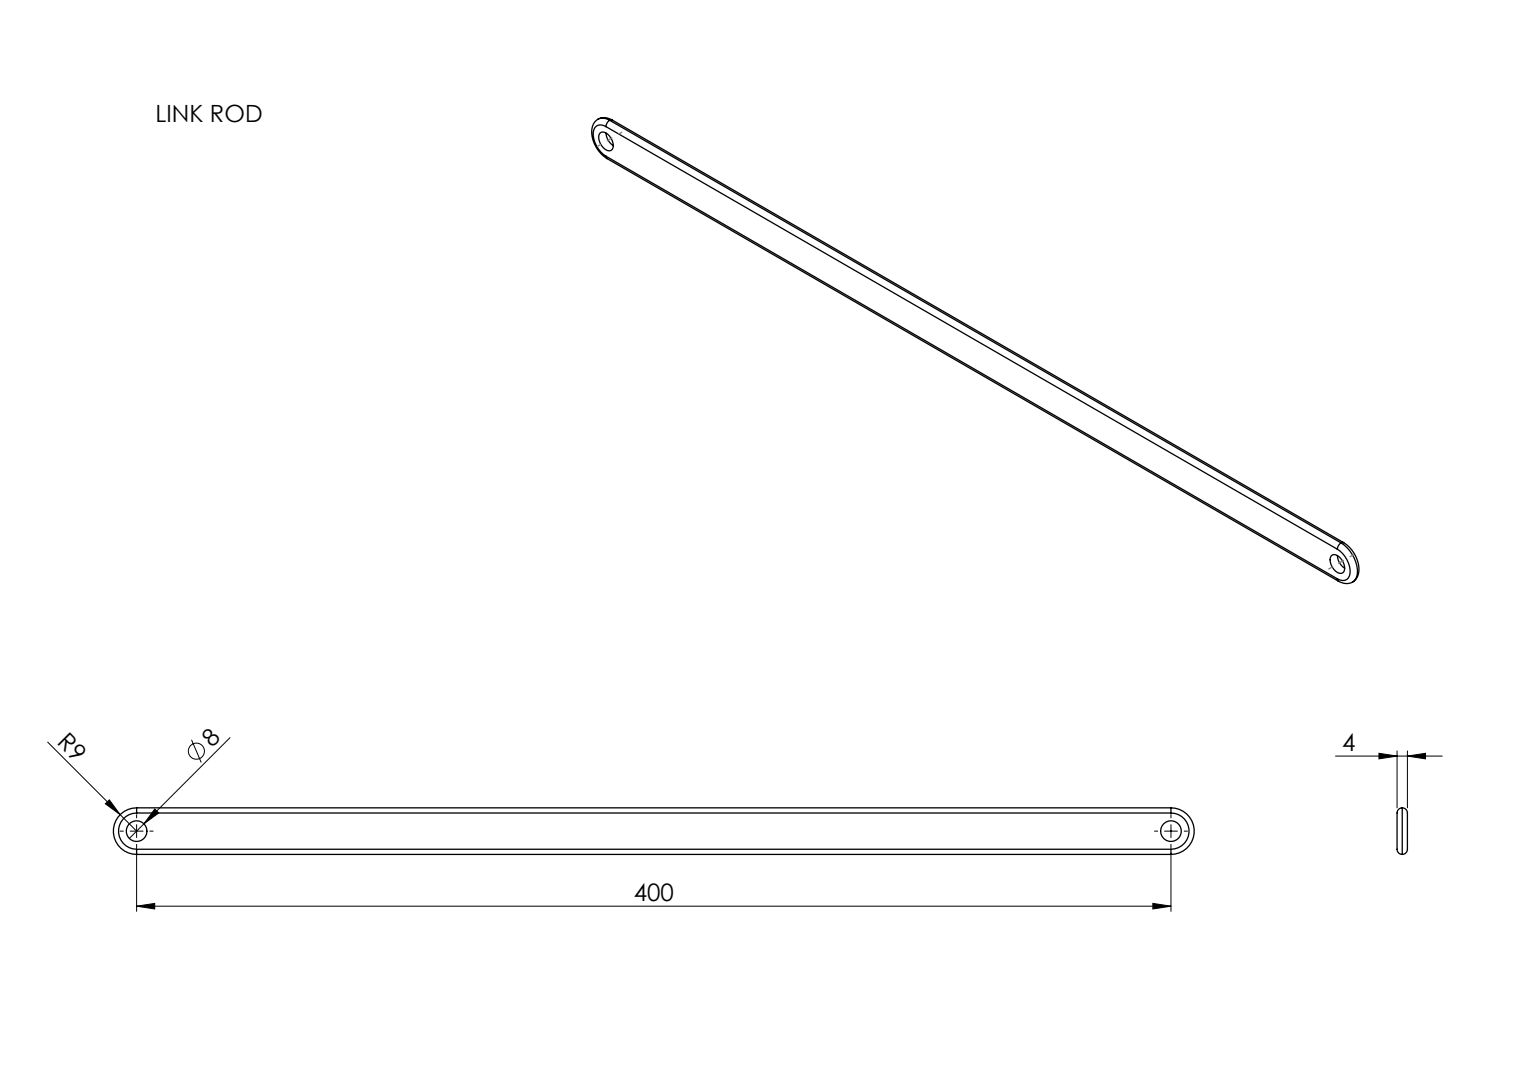
ISO-10303-21;
HEADER;
FILE_DESCRIPTION (('STEP AP214'),
    '1' );
FILE_NAME ('link rod.step',
    '2026-09-30T16:28:02',
    ( '' ),
    ( '' ),
    'SwSTEP 2.0',
    'SolidWorks 2026',
    '' );
FILE_SCHEMA (( 'AUTOMOTIVE_DESIGN' ));
ENDSEC;

DATA;
#66=CARTESIAN_POINT ( 'NONE',  ( 16.00000000000017053, 34.64101615137744972, 14.00000000000000178 ) ) ;
#129=ORIENTED_EDGE ( 'NONE', *, *, #17959, .T. ) ;
#135=ADVANCED_FACE ( 'NONE', ( #10257 ), #20396, .T. ) ;
#175=EDGE_CURVE ( 'NONE', #8969, #15955, #19420, .T. ) ;
#310=CARTESIAN_POINT ( 'NONE',  ( 20.00000000000017053, 34.64101615137744972, 14.00000000000000178 ) ) ;
#392=AXIS2_PLACEMENT_3D ( 'NONE', #4305, #4004, #27842 ) ;
#428=DIRECTION ( 'NONE',  ( -0.000000000000000000, -0.000000000000000000, -1.000000000000000000 ) ) ;
#440=AXIS2_PLACEMENT_3D ( 'NONE', #10772, #20082, #29458 ) ;
#528=( NAMED_UNIT ( * ) SI_UNIT ( $, .STERADIAN. ) SOLID_ANGLE_UNIT ( ) );
#621=CARTESIAN_POINT ( 'NONE',  ( 416.0000000000002274, 34.64101615137744972, 14.00000000000000178 ) ) ;
#662=EDGE_LOOP ( 'NONE', ( #30038, #11644, #23930, #20941 ) ) ;
#674=EDGE_LOOP ( 'NONE', ( #23723, #129, #3090, #8885 ) ) ;
#713=EDGE_CURVE ( 'NONE', #23249, #7514, #4350, .T. ) ;
#774=PRODUCT_CONTEXT ( 'NONE', #9279, 'mechanical' ) ;
#794=ORIENTED_EDGE ( 'NONE', *, *, #25575, .T. ) ;
#849=AXIS2_PLACEMENT_3D ( 'NONE', #1764, #20801, #6484 ) ;
#864=ADVANCED_FACE ( 'NONE', ( #26946 ), #28757, .T. ) ;
#870=VECTOR ( 'NONE', #18675, 1000.000000000000000 ) ;
#1083=DIRECTION ( 'NONE',  ( -0.000000000000000000, -0.000000000000000000, -1.000000000000000000 ) ) ;
#1179=DIRECTION ( 'NONE',  ( 1.000000000000000000, 0.000000000000000000, 0.000000000000000000 ) ) ;
#1186=CARTESIAN_POINT ( 'NONE',  ( 20.00000000000017053, 34.64101615137744972, 10.00000000000000178 ) ) ;
#1233=FACE_OUTER_BOUND ( 'NONE', #4292, .T. ) ;
#1344=DIRECTION ( 'NONE',  ( 1.000000000000000000, -0.000000000000000000, -0.000000000000000000 ) ) ;
#1401=DIRECTION ( 'NONE',  ( 0.000000000000000000, 0.000000000000000000, 1.000000000000000000 ) ) ;
#1402=ORIENTED_EDGE ( 'NONE', *, *, #6678, .T. ) ;
#1466=CYLINDRICAL_SURFACE ( 'NONE', #4682, 2.000000000000000000 ) ;
#1628=ADVANCED_FACE ( 'NONE', ( #7128 ), #19463, .T. ) ;
#1649=CARTESIAN_POINT ( 'NONE',  ( 20.00000000000017053, 27.64101615137744972, 12.00000000000000178 ) ) ;
#1664=ORIENTED_EDGE ( 'NONE', *, *, #12629, .T. ) ;
#1764=CARTESIAN_POINT ( 'NONE',  ( 420.0000000000002274, 34.64101615137744972, 10.00000000000000178 ) ) ;
#1776=VECTOR ( 'NONE', #11033, 1000.000000000000000 ) ;
#1792=ORIENTED_EDGE ( 'NONE', *, *, #30164, .T. ) ;
#1813=CARTESIAN_POINT ( 'NONE',  ( 416.0000000000002274, 34.64101615137744972, 10.00000000000000178 ) ) ;
#1819=ORIENTED_EDGE ( 'NONE', *, *, #20781, .T. ) ;
#1876=SURFACE_SIDE_STYLE ('',( #27386 ) ) ;
#2221=FILL_AREA_STYLE ('',( #18679 ) ) ;
#2391=AXIS2_PLACEMENT_3D ( 'NONE', #310, #18914, #21646 ) ;
#2396=ORIENTED_EDGE ( 'NONE', *, *, #11470, .T. ) ;
#2428=CARTESIAN_POINT ( 'NONE',  ( 20.00000000000017053, 34.64101615137744972, 14.00000000000000178 ) ) ;
#2445=STYLED_ITEM ( 'NONE', ( #18984 ), #16384 ) ;
#2468=PRODUCT_DEFINITION_FORMATION_WITH_SPECIFIED_SOURCE ( 'ANY', '', #20070, .NOT_KNOWN. ) ;
#2584=DIRECTION ( 'NONE',  ( 0.000000000000000000, 0.000000000000000000, 1.000000000000000000 ) ) ;
#2603=AXIS2_PLACEMENT_3D ( 'NONE', #20401, #18720, #4388 ) ;
#2609=ORIENTED_EDGE ( 'NONE', *, *, #26221, .F. ) ;
#2624=VERTEX_POINT ( 'NONE', #7362 ) ;
#2662=EDGE_LOOP ( 'NONE', ( #12047, #2609 ) ) ;
#2912=DIRECTION ( 'NONE',  ( -1.000000000000000000, 0.000000000000000000, 0.000000000000000000 ) ) ;
#3024=CARTESIAN_POINT ( 'NONE',  ( 427.0000000000002274, 34.64101615137744972, 14.00000000000000178 ) ) ;
#3081=ORIENTED_EDGE ( 'NONE', *, *, #17585, .T. ) ;
#3090=ORIENTED_EDGE ( 'NONE', *, *, #25828, .T. ) ;
#3122=CARTESIAN_POINT ( 'NONE',  ( 416.0000000000002274, 34.64101615137744972, 14.00000000000000178 ) ) ;
#3146=CARTESIAN_POINT ( 'NONE',  ( 420.0000000000002274, 34.64101615137744972, 12.00000000000000178 ) ) ;
#3242=ADVANCED_FACE ( 'NONE', ( #21504, #17633, #24672 ), #26248, .T. ) ;
#3383=DIRECTION ( 'NONE',  ( 1.000000000000000000, -0.000000000000000000, 0.000000000000000000 ) ) ;
#3440=EDGE_CURVE ( 'NONE', #8350, #23249, #13584, .T. ) ;
#3539=LINE ( 'NONE', #22146, #28159 ) ;
#3588=CARTESIAN_POINT ( 'NONE',  ( 420.0000000000002274, 34.64101615137744972, 12.00000000000000178 ) ) ;
#3601=CARTESIAN_POINT ( 'NONE',  ( 429.0000000000002274, 34.64101615137744972, 12.00000000000000178 ) ) ;
#3646=EDGE_CURVE ( 'NONE', #28740, #7514, #22998, .T. ) ;
#3694=ORIENTED_EDGE ( 'NONE', *, *, #15888, .T. ) ;
#3736=ORIENTED_EDGE ( 'NONE', *, *, #11470, .F. ) ;
#3777=DIRECTION ( 'NONE',  ( 1.000000000000000000, 0.000000000000000000, 0.000000000000000000 ) ) ;
#3861=AXIS2_PLACEMENT_3D ( 'NONE', #3146, #5571, #17603 ) ;
#4004=DIRECTION ( 'NONE',  ( 0.000000000000000000, 0.000000000000000000, 1.000000000000000000 ) ) ;
#4060=DIRECTION ( 'NONE',  ( 0.000000000000000000, 0.000000000000000000, -1.000000000000000000 ) ) ;
#4128=LINE ( 'NONE', #17840, #13960 ) ;
#4196=TOROIDAL_SURFACE ( 'NONE', #5144, 7.000000000000000888, 2.000000000000000000 ) ;
#4259=COLOUR_RGB ( '', 0.08235294, 0.09019608, 0.10196078) ;
#4292=EDGE_LOOP ( 'NONE', ( #1664, #4911, #6108, #16603 ) ) ;
#4305=CARTESIAN_POINT ( 'NONE',  ( 420.0000000000002274, 34.64101615137744972, 14.00000000000000178 ) ) ;
#4306=DIRECTION ( 'NONE',  ( 1.000000000000000000, 0.000000000000000000, 0.000000000000000000 ) ) ;
#4350=CIRCLE ( 'NONE', #3861, 9.000000000000007105 ) ;
#4388=DIRECTION ( 'NONE',  ( 0.000000000000000000, 0.000000000000000000, 1.000000000000000000 ) ) ;
#4539=DIRECTION ( 'NONE',  ( 0.000000000000000000, 0.000000000000000000, 1.000000000000000000 ) ) ;
#4541=CIRCLE ( 'NONE', #9384, 2.000000000000000000 ) ;
#4640=SHAPE_REPRESENTATION_RELATIONSHIP ( 'NONE' , 'NONE' ,  #19847, #16384 ) ;
#4682=AXIS2_PLACEMENT_3D ( 'NONE', #22519, #24507, #24965 ) ;
#4821=ORIENTED_EDGE ( 'NONE', *, *, #25575, .F. ) ;
#4904=CIRCLE ( 'NONE', #20492, 2.000000000000000000 ) ;
#4911=ORIENTED_EDGE ( 'NONE', *, *, #9408, .F. ) ;
#4940=( LENGTH_UNIT ( ) NAMED_UNIT ( * ) SI_UNIT ( .MILLI., .METRE. ) );
#4992=EDGE_LOOP ( 'NONE', ( #20045, #15327, #18477, #14680 ) ) ;
#5028=CARTESIAN_POINT ( 'NONE',  ( 20.00000000000017053, 34.64101615137744972, 14.00000000000000178 ) ) ;
#5144=AXIS2_PLACEMENT_3D ( 'NONE', #16753, #26076, #26228 ) ;
#5185=ORIENTED_EDGE ( 'NONE', *, *, #3646, .T. ) ;
#5247=VERTEX_POINT ( 'NONE', #18395 ) ;
#5272=ORIENTED_EDGE ( 'NONE', *, *, #9408, .T. ) ;
#5360=VECTOR ( 'NONE', #25155, 1000.000000000000000 ) ;
#5435=CARTESIAN_POINT ( 'NONE',  ( 0.000000000000000000, 0.000000000000000000, 0.000000000000000000 ) ) ;
#5447=DIRECTION ( 'NONE',  ( 0.000000000000000000, 0.000000000000000000, -1.000000000000000000 ) ) ;
#5537=DIRECTION ( 'NONE',  ( 1.000000000000000000, 0.000000000000000000, 0.000000000000000000 ) ) ;
#5571=DIRECTION ( 'NONE',  ( -0.000000000000000000, -0.000000000000000000, -1.000000000000000000 ) ) ;
#5577=CARTESIAN_POINT ( 'NONE',  ( 420.0000000000002274, 34.64101615137744972, 14.00000000000000178 ) ) ;
#5614=ORIENTED_EDGE ( 'NONE', *, *, #6819, .F. ) ;
#5618=VERTEX_POINT ( 'NONE', #22506 ) ;
#5628=CARTESIAN_POINT ( 'NONE',  ( 20.00000000000017053, 25.64101615137744616, 12.00000000000000178 ) ) ;
#5735=CARTESIAN_POINT ( 'NONE',  ( 20.00000000000017053, 34.64101615137744972, 10.00000000000000178 ) ) ;
#5886=EDGE_LOOP ( 'NONE', ( #16599, #6085, #10247, #2396 ) ) ;
#5903=DIRECTION ( 'NONE',  ( 1.000000000000000000, 0.000000000000000000, 0.000000000000000000 ) ) ;
#5922=ORIENTED_EDGE ( 'NONE', *, *, #25828, .F. ) ;
#6003=DIRECTION ( 'NONE',  ( 1.000000000000000000, 0.000000000000000000, 0.000000000000000000 ) ) ;
#6085=ORIENTED_EDGE ( 'NONE', *, *, #17585, .F. ) ;
#6102=ORIENTED_EDGE ( 'NONE', *, *, #9626, .T. ) ;
#6108=ORIENTED_EDGE ( 'NONE', *, *, #24279, .F. ) ;
#6142=AXIS2_PLACEMENT_3D ( 'NONE', #5028, #12042, #2912 ) ;
#6191=ADVANCED_FACE ( 'NONE', ( #10705, #13294, #15729 ), #10546, .F. ) ;
#6223=AXIS2_PLACEMENT_3D ( 'NONE', #12751, #17037, #5447 ) ;
#6248=TOROIDAL_SURFACE ( 'NONE', #13052, 7.000000000000000888, 2.000000000000000000 ) ;
#6258=VERTEX_POINT ( 'NONE', #15118 ) ;
#6275=ORIENTED_EDGE ( 'NONE', *, *, #21485, .T. ) ;
#6292=CARTESIAN_POINT ( 'NONE',  ( 20.00000000000017053, 34.64101615137744972, 12.00000000000000178 ) ) ;
#6393=DIRECTION ( 'NONE',  ( -1.000000000000000000, 0.000000000000000000, 0.000000000000000000 ) ) ;
#6484=DIRECTION ( 'NONE',  ( 1.000000000000000000, 0.000000000000000000, 0.000000000000000000 ) ) ;
#6566=DIRECTION ( 'NONE',  ( -0.000000000000000000, -0.000000000000000000, -1.000000000000000000 ) ) ;
#6678=EDGE_CURVE ( 'NONE', #7514, #9503, #6876, .T. ) ;
#6728=DIRECTION ( 'NONE',  ( -0.000000000000000000, -0.000000000000000000, -1.000000000000000000 ) ) ;
#6737=( NAMED_UNIT ( * ) SI_UNIT ( $, .STERADIAN. ) SOLID_ANGLE_UNIT ( ) );
#6770=DIRECTION ( 'NONE',  ( -1.000000000000000000, 0.000000000000000000, -0.000000000000000000 ) ) ;
#6819=EDGE_CURVE ( 'NONE', #8969, #24258, #4904, .T. ) ;
#6850=CARTESIAN_POINT ( 'NONE',  ( 24.00000000000017053, 34.64101615137744972, 10.00000000000000178 ) ) ;
#6874=DIRECTION ( 'NONE',  ( -1.000000000000000000, 0.000000000000000000, 0.000000000000000000 ) ) ;
#6876=CIRCLE ( 'NONE', #23944, 2.000000000000000000 ) ;
#6905=DIRECTION ( 'NONE',  ( 0.000000000000000000, 0.000000000000000000, 1.000000000000000000 ) ) ;
#6940=( NAMED_UNIT ( * ) PLANE_ANGLE_UNIT ( ) SI_UNIT ( $, .RADIAN. ) );
#6982=ORIENTED_EDGE ( 'NONE', *, *, #3646, .F. ) ;
#7034=EDGE_LOOP ( 'NONE', ( #15544, #8379, #5614, #28228 ) ) ;
#7111=AXIS2_PLACEMENT_3D ( 'NONE', #9110, #2584, #18740 ) ;
#7128=FACE_OUTER_BOUND ( 'NONE', #7034, .T. ) ;
#7210=CIRCLE ( 'NONE', #10130, 7.000000000000006217 ) ;
#7298=FACE_OUTER_BOUND ( 'NONE', #19832, .T. ) ;
#7334=VERTEX_POINT ( 'NONE', #13192 ) ;
#7357=ORIENTED_EDGE ( 'NONE', *, *, #25373, .T. ) ;
#7362=CARTESIAN_POINT ( 'NONE',  ( 420.0000000000002274, 27.64101615137744972, 14.00000000000000178 ) ) ;
#7514=VERTEX_POINT ( 'NONE', #3601 ) ;
#7683=AXIS2_PLACEMENT_3D ( 'NONE', #10441, #17464, #10754 ) ;
#7769=DIRECTION ( 'NONE',  ( 0.000000000000000000, 0.000000000000000000, -1.000000000000000000 ) ) ;
#7795=DIRECTION ( 'NONE',  ( -1.000000000000000000, 0.000000000000000000, 0.000000000000000000 ) ) ;
#7964=CARTESIAN_POINT ( 'NONE',  ( 20.00000000000017053, 27.64101615137744972, 10.00000000000000178 ) ) ;
#7972=DIRECTION ( 'NONE',  ( 0.000000000000000000, 0.000000000000000000, 1.000000000000000000 ) ) ;
#8107=DIRECTION ( 'NONE',  ( 1.000000000000000000, 0.000000000000000000, -0.000000000000000000 ) ) ;
#8142=CYLINDRICAL_SURFACE ( 'NONE', #21760, 2.000000000000000000 ) ;
#8147=MECHANICAL_DESIGN_GEOMETRIC_PRESENTATION_REPRESENTATION('',(#28653),#25224);
#8230=DIRECTION ( 'NONE',  ( 0.000000000000000000, 0.000000000000000000, -1.000000000000000000 ) ) ;
#8350=VERTEX_POINT ( 'NONE', #18795 ) ;
#8379=ORIENTED_EDGE ( 'NONE', *, *, #29365, .F. ) ;
#8542=EDGE_CURVE ( 'NONE', #16524, #12515, #20589, .T. ) ;
#8639=DIRECTION ( 'NONE',  ( 0.000000000000000000, 0.000000000000000000, -1.000000000000000000 ) ) ;
#8841=CARTESIAN_POINT ( 'NONE',  ( 420.0000000000002274, 34.64101615137744972, 10.00000000000000178 ) ) ;
#8874=AXIS2_PLACEMENT_3D ( 'NONE', #15740, #9009, #4306 ) ;
#8885=ORIENTED_EDGE ( 'NONE', *, *, #25484, .F. ) ;
#8909=ORIENTED_EDGE ( 'NONE', *, *, #3440, .F. ) ;
#8915=DIRECTION ( 'NONE',  ( 1.000000000000000000, 0.000000000000000000, -0.000000000000000000 ) ) ;
#8969=VERTEX_POINT ( 'NONE', #5628 ) ;
#9009=DIRECTION ( 'NONE',  ( 0.000000000000000000, 0.000000000000000000, 1.000000000000000000 ) ) ;
#9027=ORIENTED_EDGE ( 'NONE', *, *, #19612, .F. ) ;
#9058=EDGE_CURVE ( 'NONE', #13389, #15955, #4541, .T. ) ;
#9059=CARTESIAN_POINT ( 'NONE',  ( 20.00000000000017053, 27.64101615137744972, 12.00000000000000178 ) ) ;
#9110=CARTESIAN_POINT ( 'NONE',  ( 420.0000000000002274, 34.64101615137744972, 14.00000000000000178 ) ) ;
#9122=CARTESIAN_POINT ( 'NONE',  ( 420.0000000000002274, 34.64101615137744972, 12.00000000000000178 ) ) ;
#9185=LINE ( 'NONE', #13182, #22046 ) ;
#9279=APPLICATION_CONTEXT ( 'automotive_design' ) ;
#9292=ORIENTED_EDGE ( 'NONE', *, *, #26050, .T. ) ;
#9331=ADVANCED_FACE ( 'NONE', ( #18269 ), #27778, .F. ) ;
#9384=AXIS2_PLACEMENT_3D ( 'NONE', #10531, #3383, #19839 ) ;
#9408=EDGE_CURVE ( 'NONE', #5618, #15809, #22720, .T. ) ;
#9503=VERTEX_POINT ( 'NONE', #3024 ) ;
#9564=ORIENTED_EDGE ( 'NONE', *, *, #12629, .F. ) ;
#9626=EDGE_CURVE ( 'NONE', #5247, #29002, #9734, .T. ) ;
#9729=CARTESIAN_POINT ( 'NONE',  ( 20.00000000000017053, 34.64101615137744972, 12.00000000000000178 ) ) ;
#9734=CIRCLE ( 'NONE', #22414, 4.000000000000000000 ) ;
#9757=CARTESIAN_POINT ( 'NONE',  ( 424.0000000000002274, 34.64101615137744972, 14.00000000000000178 ) ) ;
#9814=SURFACE_STYLE_USAGE ( .BOTH. , #23410 ) ;
#9997=CIRCLE ( 'NONE', #11456, 2.000000000000000000 ) ;
#10130=AXIS2_PLACEMENT_3D ( 'NONE', #26774, #7972, #15131 ) ;
#10216=AXIS2_PLACEMENT_3D ( 'NONE', #2428, #428, #23315 ) ;
#10247=ORIENTED_EDGE ( 'NONE', *, *, #19312, .F. ) ;
#10257=FACE_OUTER_BOUND ( 'NONE', #13592, .T. ) ;
#10279=( GEOMETRIC_REPRESENTATION_CONTEXT ( 3 ) GLOBAL_UNCERTAINTY_ASSIGNED_CONTEXT ( ( #17738 ) ) GLOBAL_UNIT_ASSIGNED_CONTEXT ( ( #18528, #6940, #26014 ) ) REPRESENTATION_CONTEXT ( 'NONE', 'WORKASPACE' ) );
#10441=CARTESIAN_POINT ( 'NONE',  ( 420.0000000000002274, 34.64101615137744972, 14.00000000000000178 ) ) ;
#10446=DIRECTION ( 'NONE',  ( 1.000000000000000000, 0.000000000000000000, 0.000000000000000000 ) ) ;
#10460=CARTESIAN_POINT ( 'NONE',  ( 20.00000000000017053, 34.64101615137744972, 10.00000000000000178 ) ) ;
#10531=CARTESIAN_POINT ( 'NONE',  ( 20.00000000000017053, 41.64101615137744972, 12.00000000000000178 ) ) ;
#10546=PLANE ( 'NONE',  #13206 ) ;
#10550=DIRECTION ( 'NONE',  ( 0.000000000000000000, 0.000000000000000000, -1.000000000000000000 ) ) ;
#10630=EDGE_LOOP ( 'NONE', ( #18972, #27063, #17217, #5922 ) ) ;
#10705=FACE_OUTER_BOUND ( 'NONE', #19796, .T. ) ;
#10750=CIRCLE ( 'NONE', #17557, 7.000000000000006217 ) ;
#10754=DIRECTION ( 'NONE',  ( -1.000000000000000000, 0.000000000000000000, 0.000000000000000000 ) ) ;
#10772=CARTESIAN_POINT ( 'NONE',  ( 420.0000000000002274, 41.64101615137744972, 12.00000000000000178 ) ) ;
#10830=AXIS2_PLACEMENT_3D ( 'NONE', #8841, #18001, #6874 ) ;
#11033=DIRECTION ( 'NONE',  ( 1.000000000000000000, -0.000000000000000000, -0.000000000000000000 ) ) ;
#11053=ORIENTED_EDGE ( 'NONE', *, *, #8542, .T. ) ;
#11158=ORIENTED_EDGE ( 'NONE', *, *, #8542, .F. ) ;
#11164=ORIENTED_EDGE ( 'NONE', *, *, #13444, .F. ) ;
#11165=DIRECTION ( 'NONE',  ( 1.000000000000000000, 0.000000000000000000, 0.000000000000000000 ) ) ;
#11179=AXIS2_PLACEMENT_3D ( 'NONE', #18871, #4539, #13829 ) ;
#11190=ORIENTED_EDGE ( 'NONE', *, *, #15589, .F. ) ;
#11325=UNCERTAINTY_MEASURE_WITH_UNIT (LENGTH_MEASURE( 1.000000000000000082E-05 ), #15429, 'distance_accuracy_value', 'NONE');
#11356=DIRECTION ( 'NONE',  ( 1.000000000000000000, 0.000000000000000000, 0.000000000000000000 ) ) ;
#11420=CIRCLE ( 'NONE', #24592, 2.000000000000000000 ) ;
#11456=AXIS2_PLACEMENT_3D ( 'NONE', #16778, #14319, #7769 ) ;
#11470=EDGE_CURVE ( 'NONE', #13296, #8969, #9185, .T. ) ;
#11498=CARTESIAN_POINT ( 'NONE',  ( 20.00000000000017053, 34.64101615137744972, 14.00000000000000178 ) ) ;
#11540=CARTESIAN_POINT ( 'NONE',  ( 420.0000000000002274, 34.64101615137744972, 14.00000000000000178 ) ) ;
#11644=ORIENTED_EDGE ( 'NONE', *, *, #713, .F. ) ;
#11840=MANIFOLD_SOLID_BREP ( 'Fillet1', #24820 ) ;
#12042=DIRECTION ( 'NONE',  ( -0.000000000000000000, -0.000000000000000000, -1.000000000000000000 ) ) ;
#12047=ORIENTED_EDGE ( 'NONE', *, *, #25373, .F. ) ;
#12149=DIRECTION ( 'NONE',  ( -1.000000000000000000, -0.000000000000000000, 0.000000000000000000 ) ) ;
#12225=( GEOMETRIC_REPRESENTATION_CONTEXT ( 3 ) GLOBAL_UNCERTAINTY_ASSIGNED_CONTEXT ( ( #15902 ) ) GLOBAL_UNIT_ASSIGNED_CONTEXT ( ( #4940, #20959, #528 ) ) REPRESENTATION_CONTEXT ( 'NONE', 'WORKASPACE' ) );
#12276=AXIS2_PLACEMENT_3D ( 'NONE', #21982, #14943, #7795 ) ;
#12479=CIRCLE ( 'NONE', #13937, 2.000000000000000000 ) ;
#12515=VERTEX_POINT ( 'NONE', #20424 ) ;
#12629=EDGE_CURVE ( 'NONE', #15955, #15809, #16953, .T. ) ;
#12678=FACE_OUTER_BOUND ( 'NONE', #20099, .T. ) ;
#12751=CARTESIAN_POINT ( 'NONE',  ( 20.00000000000017053, 41.64101615137744972, 12.00000000000000178 ) ) ;
#12803=EDGE_LOOP ( 'NONE', ( #7357, #1819, #11158, #11164 ) ) ;
#12826=CARTESIAN_POINT ( 'NONE',  ( 420.0000000000002274, 34.64101615137744972, 12.00000000000000178 ) ) ;
#13052=AXIS2_PLACEMENT_3D ( 'NONE', #6292, #6905, #11165 ) ;
#13129=ORIENTED_EDGE ( 'NONE', *, *, #23600, .T. ) ;
#13182=CARTESIAN_POINT ( 'NONE',  ( 20.00000000000017053, 25.64101615137744616, 12.00000000000000178 ) ) ;
#13190=AXIS2_PLACEMENT_3D ( 'NONE', #5435, #19606, #10446 ) ;
#13192=CARTESIAN_POINT ( 'NONE',  ( 20.00000000000017053, 27.64101615137744972, 14.00000000000000178 ) ) ;
#13206=AXIS2_PLACEMENT_3D ( 'NONE', #19704, #29068, #8107 ) ;
#13294=FACE_BOUND ( 'NONE', #28997, .T. ) ;
#13296=VERTEX_POINT ( 'NONE', #28429 ) ;
#13389=VERTEX_POINT ( 'NONE', #23821 ) ;
#13444=EDGE_CURVE ( 'NONE', #25744, #16524, #19663, .T. ) ;
#13500=VERTEX_POINT ( 'NONE', #9757 ) ;
#13584=CIRCLE ( 'NONE', #440, 2.000000000000000000 ) ;
#13592=EDGE_LOOP ( 'NONE', ( #4821, #5185, #13129, #18549 ) ) ;
#13786=EDGE_CURVE ( 'NONE', #9503, #5618, #18801, .T. ) ;
#13829=DIRECTION ( 'NONE',  ( 1.000000000000000000, 0.000000000000000000, 0.000000000000000000 ) ) ;
#13857=DIRECTION ( 'NONE',  ( 1.000000000000000000, 0.000000000000000000, 0.000000000000000000 ) ) ;
#13937=AXIS2_PLACEMENT_3D ( 'NONE', #29223, #5537, #10550 ) ;
#13960=VECTOR ( 'NONE', #6566, 1000.000000000000000 ) ;
#13986=CYLINDRICAL_SURFACE ( 'NONE', #10216, 4.000000000000000000 ) ;
#14018=ADVANCED_FACE ( 'NONE', ( #7298 ), #4196, .T. ) ;
#14134=EDGE_CURVE ( 'NONE', #15955, #23249, #22394, .T. ) ;
#14158=DIRECTION ( 'NONE',  ( 1.000000000000000000, 0.000000000000000000, 0.000000000000000000 ) ) ;
#14303=DIRECTION ( 'NONE',  ( 0.000000000000000000, 0.000000000000000000, 1.000000000000000000 ) ) ;
#14319=DIRECTION ( 'NONE',  ( 1.000000000000000000, 0.000000000000000000, -0.000000000000000000 ) ) ;
#14418=AXIS2_PLACEMENT_3D ( 'NONE', #5577, #14858, #26965 ) ;
#14482=CIRCLE ( 'NONE', #7683, 4.000000000000003553 ) ;
#14680=ORIENTED_EDGE ( 'NONE', *, *, #15888, .F. ) ;
#14780=ADVANCED_FACE ( 'NONE', ( #26659 ), #1466, .T. ) ;
#14839=ORIENTED_EDGE ( 'NONE', *, *, #9058, .T. ) ;
#14858=DIRECTION ( 'NONE',  ( -0.000000000000000000, -0.000000000000000000, -1.000000000000000000 ) ) ;
#14943=DIRECTION ( 'NONE',  ( 0.000000000000000000, 0.000000000000000000, 1.000000000000000000 ) ) ;
#14975=ORIENTED_EDGE ( 'NONE', *, *, #26050, .F. ) ;
#15018=DIRECTION ( 'NONE',  ( 0.000000000000000000, 0.000000000000000000, 1.000000000000000000 ) ) ;
#15046=CARTESIAN_POINT ( 'NONE',  ( 420.0000000000002274, 43.64101615137744972, 12.00000000000000178 ) ) ;
#15118=CARTESIAN_POINT ( 'NONE',  ( 16.00000000000017053, 34.64101615137744972, 14.00000000000000178 ) ) ;
#15131=DIRECTION ( 'NONE',  ( 1.000000000000000000, 0.000000000000000000, 0.000000000000000000 ) ) ;
#15300=CARTESIAN_POINT ( 'NONE',  ( 20.00000000000017053, 41.64101615137744972, 10.00000000000000178 ) ) ;
#15327=ORIENTED_EDGE ( 'NONE', *, *, #26221, .T. ) ;
#15403=AXIS2_PLACEMENT_3D ( 'NONE', #3588, #24342, #21896 ) ;
#15429=( LENGTH_UNIT ( ) NAMED_UNIT ( * ) SI_UNIT ( .MILLI., .METRE. ) );
#15470=AXIS2_PLACEMENT_3D ( 'NONE', #5735, #15018, #24348 ) ;
#15530=APPLICATION_CONTEXT ( 'automotive_design' ) ;
#15544=ORIENTED_EDGE ( 'NONE', *, *, #9058, .F. ) ;
#15589=EDGE_CURVE ( 'NONE', #15809, #7334, #27446, .T. ) ;
#15598=ORIENTED_EDGE ( 'NONE', *, *, #3440, .T. ) ;
#15666=EDGE_LOOP ( 'NONE', ( #9027, #11190, #9564, #29438 ) ) ;
#15675=FACE_OUTER_BOUND ( 'NONE', #18558, .T. ) ;
#15729=FACE_BOUND ( 'NONE', #29331, .T. ) ;
#15740=CARTESIAN_POINT ( 'NONE',  ( 20.00000000000017053, 34.64101615137744972, 14.00000000000000178 ) ) ;
#15803=CARTESIAN_POINT ( 'NONE',  ( 420.0000000000002274, 43.64101615137744972, 12.00000000000000178 ) ) ;
#15809=VERTEX_POINT ( 'NONE', #23996 ) ;
#15826=CARTESIAN_POINT ( 'NONE',  ( 20.00000000000017053, 41.64101615137744972, 14.00000000000000178 ) ) ;
#15888=EDGE_CURVE ( 'NONE', #12515, #16524, #20573, .T. ) ;
#15902=UNCERTAINTY_MEASURE_WITH_UNIT (LENGTH_MEASURE( 1.000000000000000082E-05 ), #4940, 'distance_accuracy_value', 'NONE');
#15955=VERTEX_POINT ( 'NONE', #18292 ) ;
#16276=AXIS2_PLACEMENT_3D ( 'NONE', #9059, #8915, #18385 ) ;
#16277=DIRECTION ( 'NONE',  ( -0.000000000000000000, -0.000000000000000000, -1.000000000000000000 ) ) ;
#16312=CARTESIAN_POINT ( 'NONE',  ( 20.00000000000017053, 34.64101615137744972, 14.00000000000000178 ) ) ;
#16323=CARTESIAN_POINT ( 'NONE',  ( 427.0000000000002274, 34.64101615137744972, 10.00000000000000178 ) ) ;
#16380=SURFACE_STYLE_FILL_AREA ( #2221 ) ;
#16384=ADVANCED_BREP_SHAPE_REPRESENTATION ( '', ( #11840, #13190 ), #12225 ) ;
#16524=VERTEX_POINT ( 'NONE', #1813 ) ;
#16534=LINE ( 'NONE', #66, #870 ) ;
#16599=ORIENTED_EDGE ( 'NONE', *, *, #6819, .T. ) ;
#16603=ORIENTED_EDGE ( 'NONE', *, *, #14134, .F. ) ;
#16746=AXIS2_PLACEMENT_3D ( 'NONE', #11498, #25264, #11356 ) ;
#16753=CARTESIAN_POINT ( 'NONE',  ( 420.0000000000002274, 34.64101615137744972, 12.00000000000000178 ) ) ;
#16778=CARTESIAN_POINT ( 'NONE',  ( 420.0000000000002274, 27.64101615137744972, 12.00000000000000178 ) ) ;
#16845=VECTOR ( 'NONE', #1344, 1000.000000000000000 ) ;
#16880=CARTESIAN_POINT ( 'NONE',  ( 20.00000000000017053, 27.64101615137744972, 10.00000000000000178 ) ) ;
#16950=SHAPE_DEFINITION_REPRESENTATION ( #22776, #19847 ) ;
#16953=CIRCLE ( 'NONE', #6223, 2.000000000000000000 ) ;
#17037=DIRECTION ( 'NONE',  ( 1.000000000000000000, 0.000000000000000000, 0.000000000000000000 ) ) ;
#17217=ORIENTED_EDGE ( 'NONE', *, *, #9626, .F. ) ;
#17244=ADVANCED_FACE ( 'NONE', ( #15675 ), #25009, .T. ) ;
#17245=DIRECTION ( 'NONE',  ( 1.000000000000000000, 0.000000000000000000, -0.000000000000000000 ) ) ;
#17305=VECTOR ( 'NONE', #6728, 1000.000000000000000 ) ;
#17310=FACE_OUTER_BOUND ( 'NONE', #12803, .T. ) ;
#17464=DIRECTION ( 'NONE',  ( 0.000000000000000000, 0.000000000000000000, 1.000000000000000000 ) ) ;
#17492=DIRECTION ( 'NONE',  ( 1.000000000000000000, 0.000000000000000000, 0.000000000000000000 ) ) ;
#17543=AXIS2_PLACEMENT_3D ( 'NONE', #11540, #16277, #6393 ) ;
#17557=AXIS2_PLACEMENT_3D ( 'NONE', #17963, #27336, #29642 ) ;
#17575=ORIENTED_EDGE ( 'NONE', *, *, #23600, .F. ) ;
#17585=EDGE_CURVE ( 'NONE', #19419, #24258, #26208, .T. ) ;
#17601=DIRECTION ( 'NONE',  ( 0.000000000000000000, 0.000000000000000000, -1.000000000000000000 ) ) ;
#17603=DIRECTION ( 'NONE',  ( 1.000000000000000000, 0.000000000000000000, 0.000000000000000000 ) ) ;
#17633=FACE_BOUND ( 'NONE', #18471, .T. ) ;
#17738=UNCERTAINTY_MEASURE_WITH_UNIT (LENGTH_MEASURE( 1.000000000000000082E-05 ), #18528, 'distance_accuracy_value', 'NONE');
#17815=CIRCLE ( 'NONE', #15403, 9.000000000000007105 ) ;
#17840=CARTESIAN_POINT ( 'NONE',  ( 24.00000000000017053, 34.64101615137744972, 14.00000000000000178 ) ) ;
#17959=EDGE_CURVE ( 'NONE', #19510, #6258, #24554, .T. ) ;
#17963=CARTESIAN_POINT ( 'NONE',  ( 420.0000000000002274, 34.64101615137744972, 10.00000000000000178 ) ) ;
#18001=DIRECTION ( 'NONE',  ( 0.000000000000000000, 0.000000000000000000, 1.000000000000000000 ) ) ;
#18020=PRESENTATION_STYLE_ASSIGNMENT (( #20156 ) ) ;
#18166=ORIENTED_EDGE ( 'NONE', *, *, #14134, .T. ) ;
#18225=CIRCLE ( 'NONE', #18712, 4.000000000000000000 ) ;
#18263=ORIENTED_EDGE ( 'NONE', *, *, #22536, .T. ) ;
#18269=FACE_OUTER_BOUND ( 'NONE', #4992, .T. ) ;
#18292=CARTESIAN_POINT ( 'NONE',  ( 20.00000000000017053, 43.64101615137744972, 12.00000000000000178 ) ) ;
#18319=FILL_AREA_STYLE_COLOUR ( '', #4259 ) ;
#18385=DIRECTION ( 'NONE',  ( 0.000000000000000000, 0.000000000000000000, -1.000000000000000000 ) ) ;
#18395=CARTESIAN_POINT ( 'NONE',  ( 16.00000000000017053, 34.64101615137744972, 10.00000000000000178 ) ) ;
#18420=EDGE_CURVE ( 'NONE', #6258, #19510, #18225, .T. ) ;
#18459=DIRECTION ( 'NONE',  ( 0.000000000000000000, 0.000000000000000000, 1.000000000000000000 ) ) ;
#18471=EDGE_LOOP ( 'NONE', ( #24762, #26924 ) ) ;
#18477=ORIENTED_EDGE ( 'NONE', *, *, #13444, .T. ) ;
#18482=TOROIDAL_SURFACE ( 'NONE', #26293, 7.000000000000000888, 2.000000000000000000 ) ;
#18528=( LENGTH_UNIT ( ) NAMED_UNIT ( * ) SI_UNIT ( .MILLI., .METRE. ) );
#18549=ORIENTED_EDGE ( 'NONE', *, *, #19312, .T. ) ;
#18558=EDGE_LOOP ( 'NONE', ( #24502, #25017, #3736, #30026 ) ) ;
#18675=DIRECTION ( 'NONE',  ( -0.000000000000000000, -0.000000000000000000, -1.000000000000000000 ) ) ;
#18679=FILL_AREA_STYLE_COLOUR ( '', #25904 ) ;
#18712=AXIS2_PLACEMENT_3D ( 'NONE', #16312, #18459, #18757 ) ;
#18720=DIRECTION ( 'NONE',  ( -1.000000000000000000, 0.000000000000000000, 0.000000000000000000 ) ) ;
#18740=DIRECTION ( 'NONE',  ( 1.000000000000000000, 0.000000000000000000, 0.000000000000000000 ) ) ;
#18757=DIRECTION ( 'NONE',  ( 1.000000000000000000, 0.000000000000000000, 0.000000000000000000 ) ) ;
#18795=CARTESIAN_POINT ( 'NONE',  ( 420.0000000000002274, 41.64101615137744972, 10.00000000000000178 ) ) ;
#18801=CIRCLE ( 'NONE', #7111, 7.000000000000006217 ) ;
#18835=CARTESIAN_POINT ( 'NONE',  ( 24.00000000000017053, 34.64101615137744972, 14.00000000000000178 ) ) ;
#18871=CARTESIAN_POINT ( 'NONE',  ( 20.00000000000017053, 34.64101615137744972, 12.00000000000000178 ) ) ;
#18914=DIRECTION ( 'NONE',  ( 0.000000000000000000, 0.000000000000000000, 1.000000000000000000 ) ) ;
#18920=FACE_OUTER_BOUND ( 'NONE', #10630, .T. ) ;
#18972=ORIENTED_EDGE ( 'NONE', *, *, #18420, .T. ) ;
#18984=PRESENTATION_STYLE_ASSIGNMENT (( #9814 ) ) ;
#19312=EDGE_CURVE ( 'NONE', #13296, #19419, #11420, .T. ) ;
#19419=VERTEX_POINT ( 'NONE', #29760 ) ;
#19420=CIRCLE ( 'NONE', #29202, 9.000000000000001776 ) ;
#19463=TOROIDAL_SURFACE ( 'NONE', #11179, 7.000000000000000888, 2.000000000000000000 ) ;
#19510=VERTEX_POINT ( 'NONE', #18835 ) ;
#19532=CARTESIAN_POINT ( 'NONE',  ( 20.00000000000017053, 41.64101615137744972, 12.00000000000000178 ) ) ;
#19591=DIRECTION ( 'NONE',  ( 0.000000000000000000, 0.000000000000000000, -1.000000000000000000 ) ) ;
#19606=DIRECTION ( 'NONE',  ( 0.000000000000000000, 0.000000000000000000, 1.000000000000000000 ) ) ;
#19612=EDGE_CURVE ( 'NONE', #7334, #8969, #29514, .T. ) ;
#19663=LINE ( 'NONE', #621, #28712 ) ;
#19704=CARTESIAN_POINT ( 'NONE',  ( 20.00000000000017053, 34.64101615137744972, 10.00000000000000178 ) ) ;
#19796=EDGE_LOOP ( 'NONE', ( #6275, #1792, #794, #3081, #20526 ) ) ;
#19832=EDGE_LOOP ( 'NONE', ( #17575, #1402, #14975, #20307 ) ) ;
#19839=DIRECTION ( 'NONE',  ( 0.000000000000000000, 0.000000000000000000, -1.000000000000000000 ) ) ;
#19847=SHAPE_REPRESENTATION ( 'link rod', ( #13190 ), #12225 ) ;
#20045=ORIENTED_EDGE ( 'NONE', *, *, #20781, .F. ) ;
#20049=FACE_OUTER_BOUND ( 'NONE', #5886, .T. ) ;
#20070=PRODUCT ( 'link rod', 'link rod', '', ( #774 ) ) ;
#20082=DIRECTION ( 'NONE',  ( 1.000000000000000000, -0.000000000000000000, 0.000000000000000000 ) ) ;
#20099=EDGE_LOOP ( 'NONE', ( #6982, #22236, #15598, #21174 ) ) ;
#20156=SURFACE_STYLE_USAGE ( .BOTH. , #1876 ) ;
#20307=ORIENTED_EDGE ( 'NONE', *, *, #20883, .T. ) ;
#20396=TOROIDAL_SURFACE ( 'NONE', #30203, 7.000000000000000888, 2.000000000000000000 ) ;
#20401=CARTESIAN_POINT ( 'NONE',  ( 20.00000000000017053, 27.64101615137744972, 12.00000000000000178 ) ) ;
#20424=CARTESIAN_POINT ( 'NONE',  ( 424.0000000000002274, 34.64101615137744972, 10.00000000000000178 ) ) ;
#20442=EDGE_LOOP ( 'NONE', ( #14839, #18166, #8909, #27251 ) ) ;
#20449=LINE ( 'NONE', #23060, #17305 ) ;
#20459=FILL_AREA_STYLE ('',( #18319 ) ) ;
#20492=AXIS2_PLACEMENT_3D ( 'NONE', #1649, #3777, #8639 ) ;
#20526=ORIENTED_EDGE ( 'NONE', *, *, #29365, .T. ) ;
#20573=CIRCLE ( 'NONE', #12276, 4.000000000000003553 ) ;
#20589=CIRCLE ( 'NONE', #10830, 4.000000000000003553 ) ;
#20603=ORIENTED_EDGE ( 'NONE', *, *, #15589, .T. ) ;
#20781=EDGE_CURVE ( 'NONE', #13500, #12515, #20449, .T. ) ;
#20801=DIRECTION ( 'NONE',  ( -0.000000000000000000, -0.000000000000000000, -1.000000000000000000 ) ) ;
#20883=EDGE_CURVE ( 'NONE', #2624, #13296, #9997, .T. ) ;
#20941=ORIENTED_EDGE ( 'NONE', *, *, #13786, .F. ) ;
#20959=( NAMED_UNIT ( * ) PLANE_ANGLE_UNIT ( ) SI_UNIT ( $, .RADIAN. ) );
#21003=ADVANCED_FACE ( 'NONE', ( #18920 ), #28273, .F. ) ;
#21146=ORIENTED_EDGE ( 'NONE', *, *, #13786, .T. ) ;
#21174=ORIENTED_EDGE ( 'NONE', *, *, #713, .T. ) ;
#21449=CIRCLE ( 'NONE', #27825, 6.999999999999999112 ) ;
#21485=EDGE_CURVE ( 'NONE', #13389, #8350, #29260, .T. ) ;
#21504=FACE_OUTER_BOUND ( 'NONE', #30104, .T. ) ;
#21554=ADVANCED_FACE ( 'NONE', ( #20049 ), #8142, .T. ) ;
#21646=DIRECTION ( 'NONE',  ( 1.000000000000000000, 0.000000000000000000, -0.000000000000000000 ) ) ;
#21760=AXIS2_PLACEMENT_3D ( 'NONE', #27104, #26799, #17601 ) ;
#21844=DIRECTION ( 'NONE',  ( 1.000000000000000000, -0.000000000000000000, 0.000000000000000000 ) ) ;
#21856=EDGE_CURVE ( 'NONE', #19510, #29002, #4128, .T. ) ;
#21896=DIRECTION ( 'NONE',  ( 1.000000000000000000, 0.000000000000000000, 0.000000000000000000 ) ) ;
#21919=DIRECTION ( 'NONE',  ( 0.000000000000000000, 0.000000000000000000, 1.000000000000000000 ) ) ;
#21982=CARTESIAN_POINT ( 'NONE',  ( 420.0000000000002274, 34.64101615137744972, 10.00000000000000178 ) ) ;
#22045=CARTESIAN_POINT ( 'NONE',  ( 427.0000000000002274, 34.64101615137744972, 12.00000000000000178 ) ) ;
#22046=VECTOR ( 'NONE', #6770, 1000.000000000000000 ) ;
#22146=CARTESIAN_POINT ( 'NONE',  ( 420.0000000000002274, 27.64101615137744972, 14.00000000000000178 ) ) ;
#22174=CARTESIAN_POINT ( 'NONE',  ( 420.0000000000002274, 34.64101615137744972, 12.00000000000000178 ) ) ;
#22236=ORIENTED_EDGE ( 'NONE', *, *, #30164, .F. ) ;
#22394=LINE ( 'NONE', #15046, #16845 ) ;
#22414=AXIS2_PLACEMENT_3D ( 'NONE', #10460, #21919, #1179 ) ;
#22506=CARTESIAN_POINT ( 'NONE',  ( 420.0000000000002274, 41.64101615137744972, 14.00000000000000178 ) ) ;
#22519=CARTESIAN_POINT ( 'NONE',  ( 20.00000000000017053, 41.64101615137744972, 12.00000000000000178 ) ) ;
#22536=EDGE_CURVE ( 'NONE', #7334, #2624, #3539, .T. ) ;
#22634=DIRECTION ( 'NONE',  ( 0.000000000000000000, 0.000000000000000000, 1.000000000000000000 ) ) ;
#22720=LINE ( 'NONE', #15826, #5360 ) ;
#22776=PRODUCT_DEFINITION_SHAPE ( 'NONE', 'NONE',  #28218 ) ;
#22785=CIRCLE ( 'NONE', #849, 7.000000000000006217 ) ;
#22998=CIRCLE ( 'NONE', #26855, 2.000000000000000000 ) ;
#23060=CARTESIAN_POINT ( 'NONE',  ( 424.0000000000002274, 34.64101615137744972, 14.00000000000000178 ) ) ;
#23249=VERTEX_POINT ( 'NONE', #15803 ) ;
#23315=DIRECTION ( 'NONE',  ( -1.000000000000000000, 0.000000000000000000, 0.000000000000000000 ) ) ;
#23410=SURFACE_SIDE_STYLE ('',( #16380 ) ) ;
#23471=FACE_OUTER_BOUND ( 'NONE', #674, .T. ) ;
#23510=DIRECTION ( 'NONE',  ( 0.000000000000000000, -1.000000000000000000, 0.000000000000000000 ) ) ;
#23539=PRODUCT_DEFINITION_CONTEXT ( 'detailed design', #15530, 'design' ) ;
#23596=ADVANCED_FACE ( 'NONE', ( #17310 ), #26649, .F. ) ;
#23600=EDGE_CURVE ( 'NONE', #7514, #13296, #17815, .T. ) ;
#23723=ORIENTED_EDGE ( 'NONE', *, *, #21856, .F. ) ;
#23821=CARTESIAN_POINT ( 'NONE',  ( 20.00000000000017053, 41.64101615137744972, 10.00000000000000178 ) ) ;
#23930=ORIENTED_EDGE ( 'NONE', *, *, #24279, .T. ) ;
#23944=AXIS2_PLACEMENT_3D ( 'NONE', #27003, #23510, #24535 ) ;
#23996=CARTESIAN_POINT ( 'NONE',  ( 20.00000000000017053, 41.64101615137744972, 14.00000000000000178 ) ) ;
#24258=VERTEX_POINT ( 'NONE', #7964 ) ;
#24279=EDGE_CURVE ( 'NONE', #23249, #5618, #12479, .T. ) ;
#24342=DIRECTION ( 'NONE',  ( -0.000000000000000000, -0.000000000000000000, -1.000000000000000000 ) ) ;
#24348=DIRECTION ( 'NONE',  ( 1.000000000000000000, 0.000000000000000000, 0.000000000000000000 ) ) ;
#24350=ORIENTED_EDGE ( 'NONE', *, *, #25484, .T. ) ;
#24502=ORIENTED_EDGE ( 'NONE', *, *, #22536, .F. ) ;
#24507=DIRECTION ( 'NONE',  ( -1.000000000000000000, 0.000000000000000000, 0.000000000000000000 ) ) ;
#24535=DIRECTION ( 'NONE',  ( 0.000000000000000000, 0.000000000000000000, -1.000000000000000000 ) ) ;
#24537=VECTOR ( 'NONE', #12149, 1000.000000000000000 ) ;
#24554=CIRCLE ( 'NONE', #16746, 4.000000000000000000 ) ;
#24592=AXIS2_PLACEMENT_3D ( 'NONE', #24978, #5903, #4060 ) ;
#24672=FACE_BOUND ( 'NONE', #2662, .T. ) ;
#24762=ORIENTED_EDGE ( 'NONE', *, *, #18420, .F. ) ;
#24820=CLOSED_SHELL ( 'NONE', ( #135, #14018, #23596, #21003, #3242, #6191, #29121, #9331, #26187, #17244, #26509, #1628, #21554, #864, #14780, #28453 ) ) ;
#24965=DIRECTION ( 'NONE',  ( 0.000000000000000000, 0.000000000000000000, 1.000000000000000000 ) ) ;
#24978=CARTESIAN_POINT ( 'NONE',  ( 420.0000000000002274, 27.64101615137744972, 12.00000000000000178 ) ) ;
#25009=CYLINDRICAL_SURFACE ( 'NONE', #2603, 2.000000000000000000 ) ;
#25017=ORIENTED_EDGE ( 'NONE', *, *, #19612, .T. ) ;
#25155=DIRECTION ( 'NONE',  ( -1.000000000000000000, 0.000000000000000000, 0.000000000000000000 ) ) ;
#25224=( GEOMETRIC_REPRESENTATION_CONTEXT ( 3 ) GLOBAL_UNCERTAINTY_ASSIGNED_CONTEXT ( ( #11325 ) ) GLOBAL_UNIT_ASSIGNED_CONTEXT ( ( #15429, #29850, #6737 ) ) REPRESENTATION_CONTEXT ( 'NONE', 'WORKASPACE' ) );
#25264=DIRECTION ( 'NONE',  ( 0.000000000000000000, 0.000000000000000000, 1.000000000000000000 ) ) ;
#25373=EDGE_CURVE ( 'NONE', #25744, #13500, #14482, .T. ) ;
#25484=EDGE_CURVE ( 'NONE', #29002, #5247, #28678, .T. ) ;
#25575=EDGE_CURVE ( 'NONE', #28740, #19419, #22785, .T. ) ;
#25615=DIRECTION ( 'NONE',  ( -0.000000000000000000, -0.000000000000000000, -1.000000000000000000 ) ) ;
#25725=CIRCLE ( 'NONE', #392, 4.000000000000003553 ) ;
#25744=VERTEX_POINT ( 'NONE', #3122 ) ;
#25828=EDGE_CURVE ( 'NONE', #6258, #5247, #16534, .T. ) ;
#25904=COLOUR_RGB ( '', 0.08235294, 0.09019608, 0.10196078) ;
#26014=( NAMED_UNIT ( * ) SI_UNIT ( $, .STERADIAN. ) SOLID_ANGLE_UNIT ( ) );
#26050=EDGE_CURVE ( 'NONE', #2624, #9503, #7210, .T. ) ;
#26076=DIRECTION ( 'NONE',  ( 0.000000000000000000, 0.000000000000000000, 1.000000000000000000 ) ) ;
#26187=ADVANCED_FACE ( 'NONE', ( #27398 ), #6248, .T. ) ;
#26208=LINE ( 'NONE', #16880, #24537 ) ;
#26221=EDGE_CURVE ( 'NONE', #13500, #25744, #25725, .T. ) ;
#26228=DIRECTION ( 'NONE',  ( 1.000000000000000000, 0.000000000000000000, 0.000000000000000000 ) ) ;
#26248=PLANE ( 'NONE',  #2391 ) ;
#26293=AXIS2_PLACEMENT_3D ( 'NONE', #12826, #1401, #28916 ) ;
#26509=ADVANCED_FACE ( 'NONE', ( #1233 ), #26734, .T. ) ;
#26649=CYLINDRICAL_SURFACE ( 'NONE', #14418, 4.000000000000003553 ) ;
#26659=FACE_OUTER_BOUND ( 'NONE', #20442, .T. ) ;
#26734=CYLINDRICAL_SURFACE ( 'NONE', #29680, 2.000000000000000000 ) ;
#26774=CARTESIAN_POINT ( 'NONE',  ( 420.0000000000002274, 34.64101615137744972, 14.00000000000000178 ) ) ;
#26799=DIRECTION ( 'NONE',  ( 1.000000000000000000, 0.000000000000000000, 0.000000000000000000 ) ) ;
#26855=AXIS2_PLACEMENT_3D ( 'NONE', #22045, #28815, #19591 ) ;
#26924=ORIENTED_EDGE ( 'NONE', *, *, #17959, .F. ) ;
#26946=FACE_OUTER_BOUND ( 'NONE', #662, .T. ) ;
#26965=DIRECTION ( 'NONE',  ( -1.000000000000000000, 0.000000000000000000, 0.000000000000000000 ) ) ;
#27003=CARTESIAN_POINT ( 'NONE',  ( 427.0000000000002274, 34.64101615137744972, 12.00000000000000178 ) ) ;
#27063=ORIENTED_EDGE ( 'NONE', *, *, #21856, .T. ) ;
#27104=CARTESIAN_POINT ( 'NONE',  ( 20.00000000000017053, 27.64101615137744972, 12.00000000000000178 ) ) ;
#27251=ORIENTED_EDGE ( 'NONE', *, *, #21485, .F. ) ;
#27336=DIRECTION ( 'NONE',  ( -0.000000000000000000, -0.000000000000000000, -1.000000000000000000 ) ) ;
#27386=SURFACE_STYLE_FILL_AREA ( #20459 ) ;
#27398=FACE_OUTER_BOUND ( 'NONE', #15666, .T. ) ;
#27446=CIRCLE ( 'NONE', #8874, 6.999999999999999112 ) ;
#27778=CYLINDRICAL_SURFACE ( 'NONE', #17543, 4.000000000000003553 ) ;
#27825=AXIS2_PLACEMENT_3D ( 'NONE', #1186, #28687, #17492 ) ;
#27842=DIRECTION ( 'NONE',  ( -1.000000000000000000, 0.000000000000000000, 0.000000000000000000 ) ) ;
#28159=VECTOR ( 'NONE', #21844, 1000.000000000000000 ) ;
#28218=PRODUCT_DEFINITION ( 'UNKNOWN', '', #2468, #23539 ) ;
#28228=ORIENTED_EDGE ( 'NONE', *, *, #175, .T. ) ;
#28273=CYLINDRICAL_SURFACE ( 'NONE', #6142, 4.000000000000000000 ) ;
#28429=CARTESIAN_POINT ( 'NONE',  ( 420.0000000000002274, 25.64101615137744616, 12.00000000000000178 ) ) ;
#28453=ADVANCED_FACE ( 'NONE', ( #12678 ), #18482, .T. ) ;
#28653=STYLED_ITEM ( 'NONE', ( #18020 ), #11840 ) ;
#28678=CIRCLE ( 'NONE', #15470, 4.000000000000000000 ) ;
#28687=DIRECTION ( 'NONE',  ( -0.000000000000000000, -0.000000000000000000, -1.000000000000000000 ) ) ;
#28712=VECTOR ( 'NONE', #1083, 1000.000000000000000 ) ;
#28740=VERTEX_POINT ( 'NONE', #16323 ) ;
#28757=TOROIDAL_SURFACE ( 'NONE', #30226, 7.000000000000000888, 2.000000000000000000 ) ;
#28793=MECHANICAL_DESIGN_GEOMETRIC_PRESENTATION_REPRESENTATION('',(#2445),#10279);
#28815=DIRECTION ( 'NONE',  ( 0.000000000000000000, -1.000000000000000000, 0.000000000000000000 ) ) ;
#28916=DIRECTION ( 'NONE',  ( 1.000000000000000000, 0.000000000000000000, 0.000000000000000000 ) ) ;
#28997=EDGE_LOOP ( 'NONE', ( #6102, #24350 ) ) ;
#29002=VERTEX_POINT ( 'NONE', #6850 ) ;
#29068=DIRECTION ( 'NONE',  ( 0.000000000000000000, 0.000000000000000000, 1.000000000000000000 ) ) ;
#29121=ADVANCED_FACE ( 'NONE', ( #23471 ), #13986, .F. ) ;
#29202=AXIS2_PLACEMENT_3D ( 'NONE', #9729, #25615, #13857 ) ;
#29223=CARTESIAN_POINT ( 'NONE',  ( 420.0000000000002274, 41.64101615137744972, 12.00000000000000178 ) ) ;
#29260=LINE ( 'NONE', #15300, #1776 ) ;
#29331=EDGE_LOOP ( 'NONE', ( #11053, #3694 ) ) ;
#29365=EDGE_CURVE ( 'NONE', #24258, #13389, #21449, .T. ) ;
#29438=ORIENTED_EDGE ( 'NONE', *, *, #175, .F. ) ;
#29458=DIRECTION ( 'NONE',  ( 0.000000000000000000, 0.000000000000000000, -1.000000000000000000 ) ) ;
#29514=CIRCLE ( 'NONE', #16276, 2.000000000000000000 ) ;
#29642=DIRECTION ( 'NONE',  ( 1.000000000000000000, 0.000000000000000000, 0.000000000000000000 ) ) ;
#29680=AXIS2_PLACEMENT_3D ( 'NONE', #19532, #17245, #8230 ) ;
#29760=CARTESIAN_POINT ( 'NONE',  ( 420.0000000000002274, 27.64101615137744972, 10.00000000000000178 ) ) ;
#29850=( NAMED_UNIT ( * ) PLANE_ANGLE_UNIT ( ) SI_UNIT ( $, .RADIAN. ) );
#30026=ORIENTED_EDGE ( 'NONE', *, *, #20883, .F. ) ;
#30038=ORIENTED_EDGE ( 'NONE', *, *, #6678, .F. ) ;
#30104=EDGE_LOOP ( 'NONE', ( #18263, #9292, #21146, #5272, #20603 ) ) ;
#30164=EDGE_CURVE ( 'NONE', #8350, #28740, #10750, .T. ) ;
#30203=AXIS2_PLACEMENT_3D ( 'NONE', #9122, #14303, #14158 ) ;
#30226=AXIS2_PLACEMENT_3D ( 'NONE', #22174, #22634, #6003 ) ;
ENDSEC;
END-ISO-10303-21;
